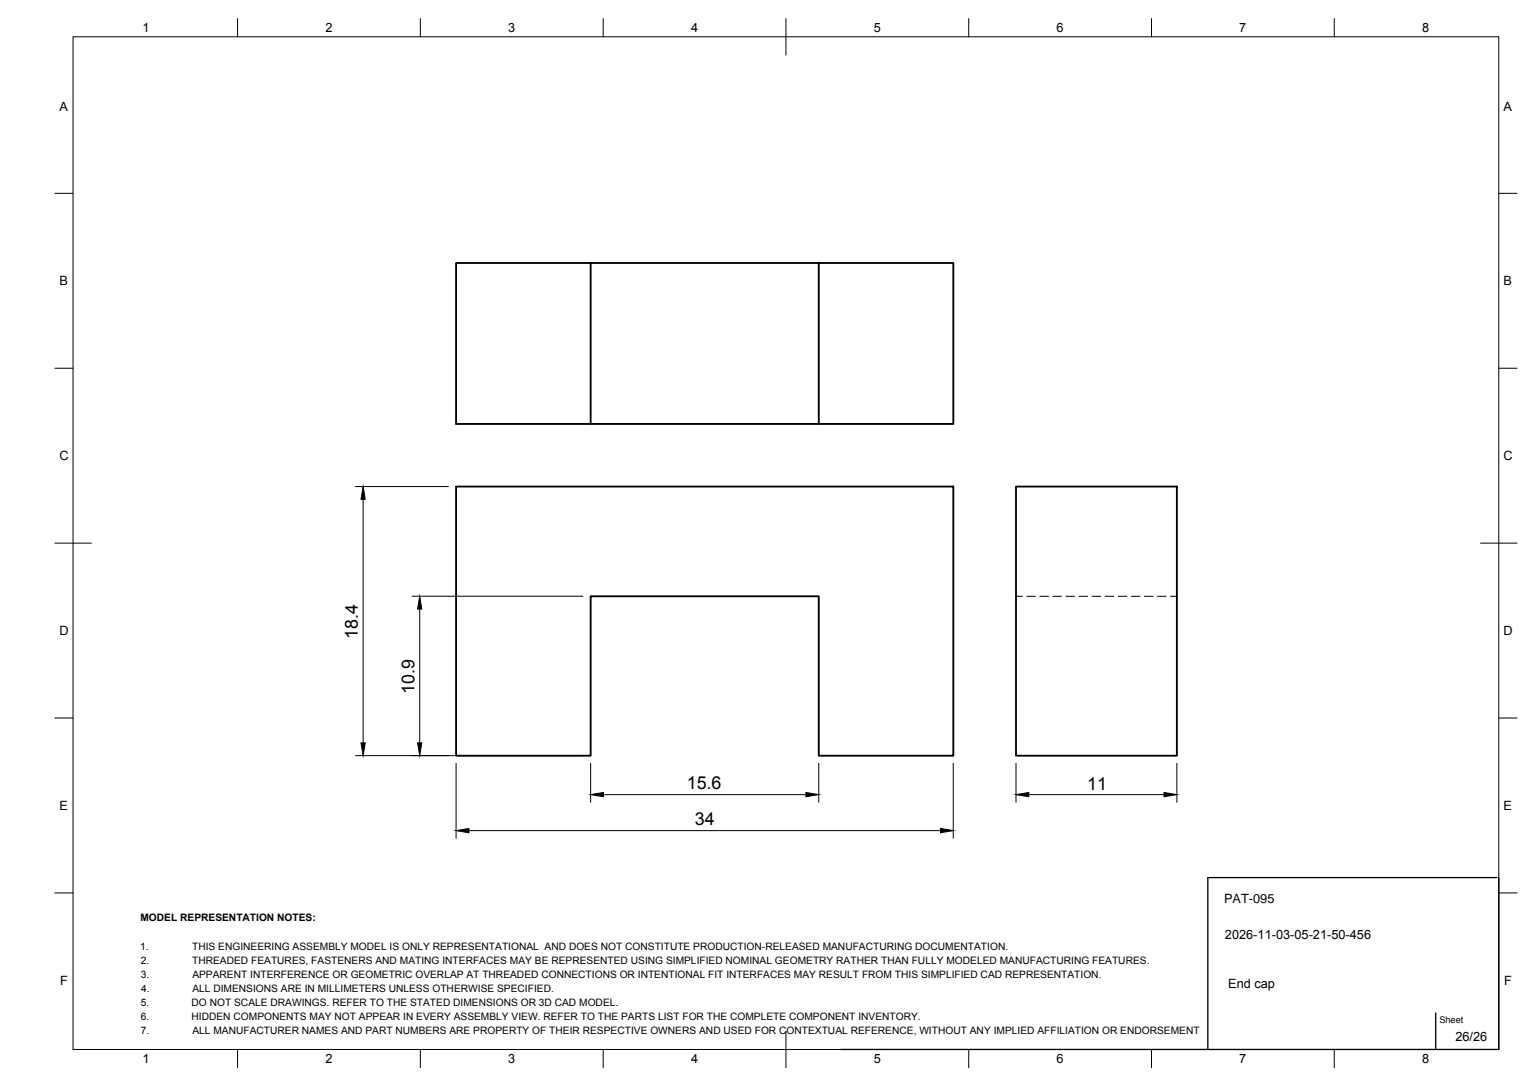
ISO-10303-21;
HEADER;
/* Generated by software containing ST-Developer
 * from STEP Tools, Inc. (www.steptools.com) 
 */

FILE_DESCRIPTION(
/* description */ ('Single-Axis Profile-Rail Linear Slide'),
/* implementation_level */ '2;1');

FILE_NAME(
/* name */ 'End cap.step',
/* time_stamp */ '2026-10-27T10:47:43-07:00',
/* author */ (''),
/* organization */ (''),
/* preprocessor_version */ 'ST-DEVELOPER v20.2',
/* originating_system */ 'Autodesk Translation Framework v15.17.0.0',
/* authorisation */ '');

FILE_SCHEMA (('AUTOMOTIVE_DESIGN { 1 0 10303 214 3 1 1 }'));
ENDSEC;

DATA;
#10=MECHANICAL_DESIGN_GEOMETRIC_PRESENTATION_REPRESENTATION('',(#349),#14478);
#295=SHAPE_REPRESENTATION_RELATIONSHIP('SRR','None',#14627,#322);
#322=ADVANCED_BREP_SHAPE_REPRESENTATION('',(#374),#14471);
#349=STYLED_ITEM('',(#14845),#374);
#374=MANIFOLD_SOLID_BREP('Body1',#8611);
#791=PLANE('',#9444);
#792=PLANE('',#9445);
#793=PLANE('',#9446);
#794=PLANE('',#9447);
#795=PLANE('',#9448);
#796=PLANE('',#9449);
#797=PLANE('',#9450);
#798=PLANE('',#9451);
#799=PLANE('',#9452);
#800=PLANE('',#9453);
#1220=FACE_OUTER_BOUND('',#1756,.T.);
#1221=FACE_OUTER_BOUND('',#1757,.T.);
#1222=FACE_OUTER_BOUND('',#1758,.T.);
#1223=FACE_OUTER_BOUND('',#1759,.T.);
#1224=FACE_OUTER_BOUND('',#1760,.T.);
#1225=FACE_OUTER_BOUND('',#1761,.T.);
#1226=FACE_OUTER_BOUND('',#1762,.T.);
#1227=FACE_OUTER_BOUND('',#1763,.T.);
#1228=FACE_OUTER_BOUND('',#1764,.T.);
#1229=FACE_OUTER_BOUND('',#1765,.T.);
#1756=EDGE_LOOP('',(#7787,#7788,#7789,#7790));
#1757=EDGE_LOOP('',(#7791,#7792,#7793,#7794));
#1758=EDGE_LOOP('',(#7795,#7796,#7797,#7798));
#1759=EDGE_LOOP('',(#7799,#7800,#7801,#7802));
#1760=EDGE_LOOP('',(#7803,#7804,#7805,#7806));
#1761=EDGE_LOOP('',(#7807,#7808,#7809,#7810));
#1762=EDGE_LOOP('',(#7811,#7812,#7813,#7814));
#1763=EDGE_LOOP('',(#7815,#7816,#7817,#7818));
#1764=EDGE_LOOP('',(#7819,#7820,#7821,#7822,#7823,#7824,#7825,#7826));
#1765=EDGE_LOOP('',(#7827,#7828,#7829,#7830,#7831,#7832,#7833,#7834));
#2707=LINE('',#14047,#3678);
#2708=LINE('',#14049,#3679);
#2709=LINE('',#14051,#3680);
#2710=LINE('',#14052,#3681);
#2711=LINE('',#14055,#3682);
#2712=LINE('',#14057,#3683);
#2713=LINE('',#14058,#3684);
#2714=LINE('',#14061,#3685);
#2715=LINE('',#14063,#3686);
#2716=LINE('',#14064,#3687);
#2717=LINE('',#14067,#3688);
#2718=LINE('',#14069,#3689);
#2719=LINE('',#14070,#3690);
#2720=LINE('',#14073,#3691);
#2721=LINE('',#14075,#3692);
#2722=LINE('',#14076,#3693);
#2723=LINE('',#14079,#3694);
#2724=LINE('',#14081,#3695);
#2725=LINE('',#14082,#3696);
#2726=LINE('',#14085,#3697);
#2727=LINE('',#14087,#3698);
#2728=LINE('',#14088,#3699);
#2729=LINE('',#14090,#3700);
#2730=LINE('',#14091,#3701);
#3678=VECTOR('',#11540,1.);
#3679=VECTOR('',#11541,1.);
#3680=VECTOR('',#11542,1.);
#3681=VECTOR('',#11543,1.);
#3682=VECTOR('',#11546,1.);
#3683=VECTOR('',#11547,1.);
#3684=VECTOR('',#11548,1.);
#3685=VECTOR('',#11551,1.);
#3686=VECTOR('',#11552,1.);
#3687=VECTOR('',#11553,1.);
#3688=VECTOR('',#11556,1.);
#3689=VECTOR('',#11557,1.);
#3690=VECTOR('',#11558,1.);
#3691=VECTOR('',#11561,1.);
#3692=VECTOR('',#11562,1.);
#3693=VECTOR('',#11563,1.);
#3694=VECTOR('',#11566,1.);
#3695=VECTOR('',#11567,1.);
#3696=VECTOR('',#11568,1.);
#3697=VECTOR('',#11571,1.);
#3698=VECTOR('',#11572,1.);
#3699=VECTOR('',#11573,1.);
#3700=VECTOR('',#11576,1.);
#3701=VECTOR('',#11577,1.);
#4594=VERTEX_POINT('',#14045);
#4595=VERTEX_POINT('',#14046);
#4596=VERTEX_POINT('',#14048);
#4597=VERTEX_POINT('',#14050);
#4598=VERTEX_POINT('',#14054);
#4599=VERTEX_POINT('',#14056);
#4600=VERTEX_POINT('',#14060);
#4601=VERTEX_POINT('',#14062);
#4602=VERTEX_POINT('',#14066);
#4603=VERTEX_POINT('',#14068);
#4604=VERTEX_POINT('',#14072);
#4605=VERTEX_POINT('',#14074);
#4606=VERTEX_POINT('',#14078);
#4607=VERTEX_POINT('',#14080);
#4608=VERTEX_POINT('',#14084);
#4609=VERTEX_POINT('',#14086);
#5671=EDGE_CURVE('',#4594,#4595,#2707,.T.);
#5672=EDGE_CURVE('',#4594,#4596,#2708,.T.);
#5673=EDGE_CURVE('',#4597,#4596,#2709,.T.);
#5674=EDGE_CURVE('',#4595,#4597,#2710,.T.);
#5675=EDGE_CURVE('',#4595,#4598,#2711,.T.);
#5676=EDGE_CURVE('',#4599,#4597,#2712,.T.);
#5677=EDGE_CURVE('',#4598,#4599,#2713,.T.);
#5678=EDGE_CURVE('',#4598,#4600,#2714,.T.);
#5679=EDGE_CURVE('',#4601,#4599,#2715,.T.);
#5680=EDGE_CURVE('',#4600,#4601,#2716,.T.);
#5681=EDGE_CURVE('',#4600,#4602,#2717,.T.);
#5682=EDGE_CURVE('',#4603,#4601,#2718,.T.);
#5683=EDGE_CURVE('',#4602,#4603,#2719,.T.);
#5684=EDGE_CURVE('',#4602,#4604,#2720,.T.);
#5685=EDGE_CURVE('',#4605,#4603,#2721,.T.);
#5686=EDGE_CURVE('',#4604,#4605,#2722,.T.);
#5687=EDGE_CURVE('',#4604,#4606,#2723,.T.);
#5688=EDGE_CURVE('',#4607,#4605,#2724,.T.);
#5689=EDGE_CURVE('',#4606,#4607,#2725,.T.);
#5690=EDGE_CURVE('',#4606,#4608,#2726,.T.);
#5691=EDGE_CURVE('',#4609,#4607,#2727,.T.);
#5692=EDGE_CURVE('',#4608,#4609,#2728,.T.);
#5693=EDGE_CURVE('',#4608,#4594,#2729,.T.);
#5694=EDGE_CURVE('',#4596,#4609,#2730,.T.);
#7787=ORIENTED_EDGE('',*,*,#5671,.F.);
#7788=ORIENTED_EDGE('',*,*,#5672,.T.);
#7789=ORIENTED_EDGE('',*,*,#5673,.F.);
#7790=ORIENTED_EDGE('',*,*,#5674,.F.);
#7791=ORIENTED_EDGE('',*,*,#5675,.F.);
#7792=ORIENTED_EDGE('',*,*,#5674,.T.);
#7793=ORIENTED_EDGE('',*,*,#5676,.F.);
#7794=ORIENTED_EDGE('',*,*,#5677,.F.);
#7795=ORIENTED_EDGE('',*,*,#5678,.F.);
#7796=ORIENTED_EDGE('',*,*,#5677,.T.);
#7797=ORIENTED_EDGE('',*,*,#5679,.F.);
#7798=ORIENTED_EDGE('',*,*,#5680,.F.);
#7799=ORIENTED_EDGE('',*,*,#5681,.F.);
#7800=ORIENTED_EDGE('',*,*,#5680,.T.);
#7801=ORIENTED_EDGE('',*,*,#5682,.F.);
#7802=ORIENTED_EDGE('',*,*,#5683,.F.);
#7803=ORIENTED_EDGE('',*,*,#5684,.F.);
#7804=ORIENTED_EDGE('',*,*,#5683,.T.);
#7805=ORIENTED_EDGE('',*,*,#5685,.F.);
#7806=ORIENTED_EDGE('',*,*,#5686,.F.);
#7807=ORIENTED_EDGE('',*,*,#5687,.F.);
#7808=ORIENTED_EDGE('',*,*,#5686,.T.);
#7809=ORIENTED_EDGE('',*,*,#5688,.F.);
#7810=ORIENTED_EDGE('',*,*,#5689,.F.);
#7811=ORIENTED_EDGE('',*,*,#5690,.F.);
#7812=ORIENTED_EDGE('',*,*,#5689,.T.);
#7813=ORIENTED_EDGE('',*,*,#5691,.F.);
#7814=ORIENTED_EDGE('',*,*,#5692,.F.);
#7815=ORIENTED_EDGE('',*,*,#5693,.F.);
#7816=ORIENTED_EDGE('',*,*,#5692,.T.);
#7817=ORIENTED_EDGE('',*,*,#5694,.F.);
#7818=ORIENTED_EDGE('',*,*,#5672,.F.);
#7819=ORIENTED_EDGE('',*,*,#5693,.T.);
#7820=ORIENTED_EDGE('',*,*,#5671,.T.);
#7821=ORIENTED_EDGE('',*,*,#5675,.T.);
#7822=ORIENTED_EDGE('',*,*,#5678,.T.);
#7823=ORIENTED_EDGE('',*,*,#5681,.T.);
#7824=ORIENTED_EDGE('',*,*,#5684,.T.);
#7825=ORIENTED_EDGE('',*,*,#5687,.T.);
#7826=ORIENTED_EDGE('',*,*,#5690,.T.);
#7827=ORIENTED_EDGE('',*,*,#5694,.T.);
#7828=ORIENTED_EDGE('',*,*,#5691,.T.);
#7829=ORIENTED_EDGE('',*,*,#5688,.T.);
#7830=ORIENTED_EDGE('',*,*,#5685,.T.);
#7831=ORIENTED_EDGE('',*,*,#5682,.T.);
#7832=ORIENTED_EDGE('',*,*,#5679,.T.);
#7833=ORIENTED_EDGE('',*,*,#5676,.T.);
#7834=ORIENTED_EDGE('',*,*,#5673,.T.);
#8514=ADVANCED_FACE('',(#1220),#791,.T.);
#8515=ADVANCED_FACE('',(#1221),#792,.T.);
#8516=ADVANCED_FACE('',(#1222),#793,.T.);
#8517=ADVANCED_FACE('',(#1223),#794,.T.);
#8518=ADVANCED_FACE('',(#1224),#795,.T.);
#8519=ADVANCED_FACE('',(#1225),#796,.T.);
#8520=ADVANCED_FACE('',(#1226),#797,.T.);
#8521=ADVANCED_FACE('',(#1227),#798,.T.);
#8522=ADVANCED_FACE('',(#1228),#799,.T.);
#8523=ADVANCED_FACE('',(#1229),#800,.T.);
#8611=CLOSED_SHELL('',(#8514,#8515,#8516,#8517,#8518,#8519,#8520,#8521,
#8522,#8523));
#9443=AXIS2_PLACEMENT_3D('',#14043,#11536,#11537);
#9444=AXIS2_PLACEMENT_3D('',#14044,#11538,#11539);
#9445=AXIS2_PLACEMENT_3D('',#14053,#11544,#11545);
#9446=AXIS2_PLACEMENT_3D('',#14059,#11549,#11550);
#9447=AXIS2_PLACEMENT_3D('',#14065,#11554,#11555);
#9448=AXIS2_PLACEMENT_3D('',#14071,#11559,#11560);
#9449=AXIS2_PLACEMENT_3D('',#14077,#11564,#11565);
#9450=AXIS2_PLACEMENT_3D('',#14083,#11569,#11570);
#9451=AXIS2_PLACEMENT_3D('',#14089,#11574,#11575);
#9452=AXIS2_PLACEMENT_3D('',#14092,#11578,#11579);
#9453=AXIS2_PLACEMENT_3D('',#14093,#11580,#11581);
#11536=DIRECTION('axis',(0.,0.,1.));
#11537=DIRECTION('refdir',(1.,0.,0.));
#11538=DIRECTION('center_axis',(0.,0.,-1.));
#11539=DIRECTION('ref_axis',(0.,-1.,0.));
#11540=DIRECTION('',(0.,1.,0.));
#11541=DIRECTION('',(-1.,0.,0.));
#11542=DIRECTION('',(0.,-1.,0.));
#11543=DIRECTION('',(-1.,0.,0.));
#11544=DIRECTION('center_axis',(0.,1.,0.));
#11545=DIRECTION('ref_axis',(0.,0.,-1.));
#11546=DIRECTION('',(0.,0.,1.));
#11547=DIRECTION('',(0.,0.,-1.));
#11548=DIRECTION('',(-1.,0.,0.));
#11549=DIRECTION('center_axis',(0.,0.,-1.));
#11550=DIRECTION('ref_axis',(0.,-1.,0.));
#11551=DIRECTION('',(0.,1.,0.));
#11552=DIRECTION('',(0.,-1.,0.));
#11553=DIRECTION('',(-1.,0.,0.));
#11554=DIRECTION('center_axis',(0.,-1.,0.));
#11555=DIRECTION('ref_axis',(0.,0.,1.));
#11556=DIRECTION('',(0.,0.,-1.));
#11557=DIRECTION('',(0.,0.,1.));
#11558=DIRECTION('',(-1.,0.,0.));
#11559=DIRECTION('center_axis',(0.,0.,-1.));
#11560=DIRECTION('ref_axis',(0.,-1.,0.));
#11561=DIRECTION('',(0.,1.,0.));
#11562=DIRECTION('',(0.,-1.,0.));
#11563=DIRECTION('',(-1.,0.,0.));
#11564=DIRECTION('center_axis',(0.,1.,0.));
#11565=DIRECTION('ref_axis',(0.,0.,-1.));
#11566=DIRECTION('',(0.,0.,1.));
#11567=DIRECTION('',(0.,0.,-1.));
#11568=DIRECTION('',(-1.,0.,0.));
#11569=DIRECTION('center_axis',(0.,0.,1.));
#11570=DIRECTION('ref_axis',(0.,1.,0.));
#11571=DIRECTION('',(0.,-1.,0.));
#11572=DIRECTION('',(0.,1.,0.));
#11573=DIRECTION('',(-1.,0.,0.));
#11574=DIRECTION('center_axis',(0.,-1.,0.));
#11575=DIRECTION('ref_axis',(0.,0.,1.));
#11576=DIRECTION('',(0.,0.,-1.));
#11577=DIRECTION('',(0.,0.,1.));
#11578=DIRECTION('center_axis',(1.,0.,0.));
#11579=DIRECTION('ref_axis',(0.,0.,-1.));
#11580=DIRECTION('center_axis',(-1.,0.,0.));
#11581=DIRECTION('ref_axis',(0.,0.,1.));
#14043=CARTESIAN_POINT('',(0.,0.,0.));
#14044=CARTESIAN_POINT('Origin',(-1.97,-0.78,0.46));
#14045=CARTESIAN_POINT('',(-1.97,-1.7,0.46));
#14046=CARTESIAN_POINT('',(-1.97,-0.78,0.46));
#14047=CARTESIAN_POINT('',(-1.97,-1.7,0.46));
#14048=CARTESIAN_POINT('',(-3.07,-1.7,0.46));
#14049=CARTESIAN_POINT('',(-1.97,-1.7,0.46));
#14050=CARTESIAN_POINT('',(-3.07,-0.78,0.46));
#14051=CARTESIAN_POINT('',(-3.07,-1.7,0.46));
#14052=CARTESIAN_POINT('',(-1.97,-0.78,0.46));
#14053=CARTESIAN_POINT('Origin',(-1.97,-0.78,1.55));
#14054=CARTESIAN_POINT('',(-1.97,-0.78,1.55));
#14055=CARTESIAN_POINT('',(-1.97,-0.78,0.46));
#14056=CARTESIAN_POINT('',(-3.07,-0.78,1.55));
#14057=CARTESIAN_POINT('',(-3.07,-0.78,0.46));
#14058=CARTESIAN_POINT('',(-1.97,-0.78,1.55));
#14059=CARTESIAN_POINT('Origin',(-1.97,0.78,1.55));
#14060=CARTESIAN_POINT('',(-1.97,0.78,1.55));
#14061=CARTESIAN_POINT('',(-1.97,-0.78,1.55));
#14062=CARTESIAN_POINT('',(-3.07,0.78,1.55));
#14063=CARTESIAN_POINT('',(-3.07,-0.78,1.55));
#14064=CARTESIAN_POINT('',(-1.97,0.78,1.55));
#14065=CARTESIAN_POINT('Origin',(-1.97,0.78,0.46));
#14066=CARTESIAN_POINT('',(-1.97,0.78,0.46));
#14067=CARTESIAN_POINT('',(-1.97,0.78,1.55));
#14068=CARTESIAN_POINT('',(-3.07,0.78,0.46));
#14069=CARTESIAN_POINT('',(-3.07,0.78,1.55));
#14070=CARTESIAN_POINT('',(-1.97,0.78,0.46));
#14071=CARTESIAN_POINT('Origin',(-1.97,1.7,0.46));
#14072=CARTESIAN_POINT('',(-1.97,1.7,0.46));
#14073=CARTESIAN_POINT('',(-1.97,0.78,0.46));
#14074=CARTESIAN_POINT('',(-3.07,1.7,0.46));
#14075=CARTESIAN_POINT('',(-3.07,0.78,0.46));
#14076=CARTESIAN_POINT('',(-1.97,1.7,0.46));
#14077=CARTESIAN_POINT('Origin',(-1.97,1.7,2.3));
#14078=CARTESIAN_POINT('',(-1.97,1.7,2.3));
#14079=CARTESIAN_POINT('',(-1.97,1.7,0.46));
#14080=CARTESIAN_POINT('',(-3.07,1.7,2.3));
#14081=CARTESIAN_POINT('',(-3.07,1.7,0.46));
#14082=CARTESIAN_POINT('',(-1.97,1.7,2.3));
#14083=CARTESIAN_POINT('Origin',(-1.97,-1.7,2.3));
#14084=CARTESIAN_POINT('',(-1.97,-1.7,2.3));
#14085=CARTESIAN_POINT('',(-1.97,1.7,2.3));
#14086=CARTESIAN_POINT('',(-3.07,-1.7,2.3));
#14087=CARTESIAN_POINT('',(-3.07,1.7,2.3));
#14088=CARTESIAN_POINT('',(-1.97,-1.7,2.3));
#14089=CARTESIAN_POINT('Origin',(-1.97,-1.7,0.46));
#14090=CARTESIAN_POINT('',(-1.97,-1.7,2.3));
#14091=CARTESIAN_POINT('',(-3.07,-1.7,2.3));
#14092=CARTESIAN_POINT('Origin',(-1.97,0.,1.38));
#14093=CARTESIAN_POINT('Origin',(-3.07,0.,1.38));
#14439=UNCERTAINTY_MEASURE_WITH_UNIT(LENGTH_MEASURE(0.001),#14479,
'DISTANCE_ACCURACY_VALUE',
'Maximum model space distance between geometric entities at asserted c
onnectivities');
#14446=UNCERTAINTY_MEASURE_WITH_UNIT(LENGTH_MEASURE(0.001),#14479,
'DISTANCE_ACCURACY_VALUE',
'Maximum model space distance between geometric entities at asserted c
onnectivities');
#14471=(
GEOMETRIC_REPRESENTATION_CONTEXT(3)
GLOBAL_UNCERTAINTY_ASSIGNED_CONTEXT((#14439))
GLOBAL_UNIT_ASSIGNED_CONTEXT((#14479,#14481,#14482))
REPRESENTATION_CONTEXT('','3D')
);
#14478=(
GEOMETRIC_REPRESENTATION_CONTEXT(3)
GLOBAL_UNCERTAINTY_ASSIGNED_CONTEXT((#14446))
GLOBAL_UNIT_ASSIGNED_CONTEXT((#14479,#14481,#14482))
REPRESENTATION_CONTEXT('','3D')
);
#14479=(
LENGTH_UNIT()
NAMED_UNIT(*)
SI_UNIT(.CENTI.,.METRE.)
);
#14481=(
NAMED_UNIT(*)
PLANE_ANGLE_UNIT()
SI_UNIT($,.RADIAN.)
);
#14482=(
NAMED_UNIT(*)
SI_UNIT($,.STERADIAN.)
SOLID_ANGLE_UNIT()
);
#14507=SHAPE_DEFINITION_REPRESENTATION(#14538,#14627);
#14538=PRODUCT_DEFINITION_SHAPE('',$,#14659);
#14627=SHAPE_REPRESENTATION('',(#9443),#14471);
#14634=PRODUCT_DEFINITION_CONTEXT('part definition',#14729,'design');
#14659=PRODUCT_DEFINITION('End cap','End cap',#14690,#14634);
#14690=PRODUCT_DEFINITION_FORMATION('',$,#14755);
#14729=APPLICATION_CONTEXT(
'Core Data for Automotive Mechanical Design Process');
#14730=PRODUCT_CONTEXT('part definition',#14729,'mechanical');
#14755=PRODUCT('End cap','End cap','End cap',(#14730));
#14839=COLOUR_RGB('Off White',0.89,0.88,0.83);
#14840=FILL_AREA_STYLE_COLOUR('',#14839);
#14841=FILL_AREA_STYLE('',(#14840));
#14842=SURFACE_STYLE_FILL_AREA(#14841);
#14843=SURFACE_SIDE_STYLE('',(#14842));
#14844=SURFACE_STYLE_USAGE(.BOTH.,#14843);
#14845=PRESENTATION_STYLE_ASSIGNMENT((#14844));
ENDSEC;
END-ISO-10303-21;
